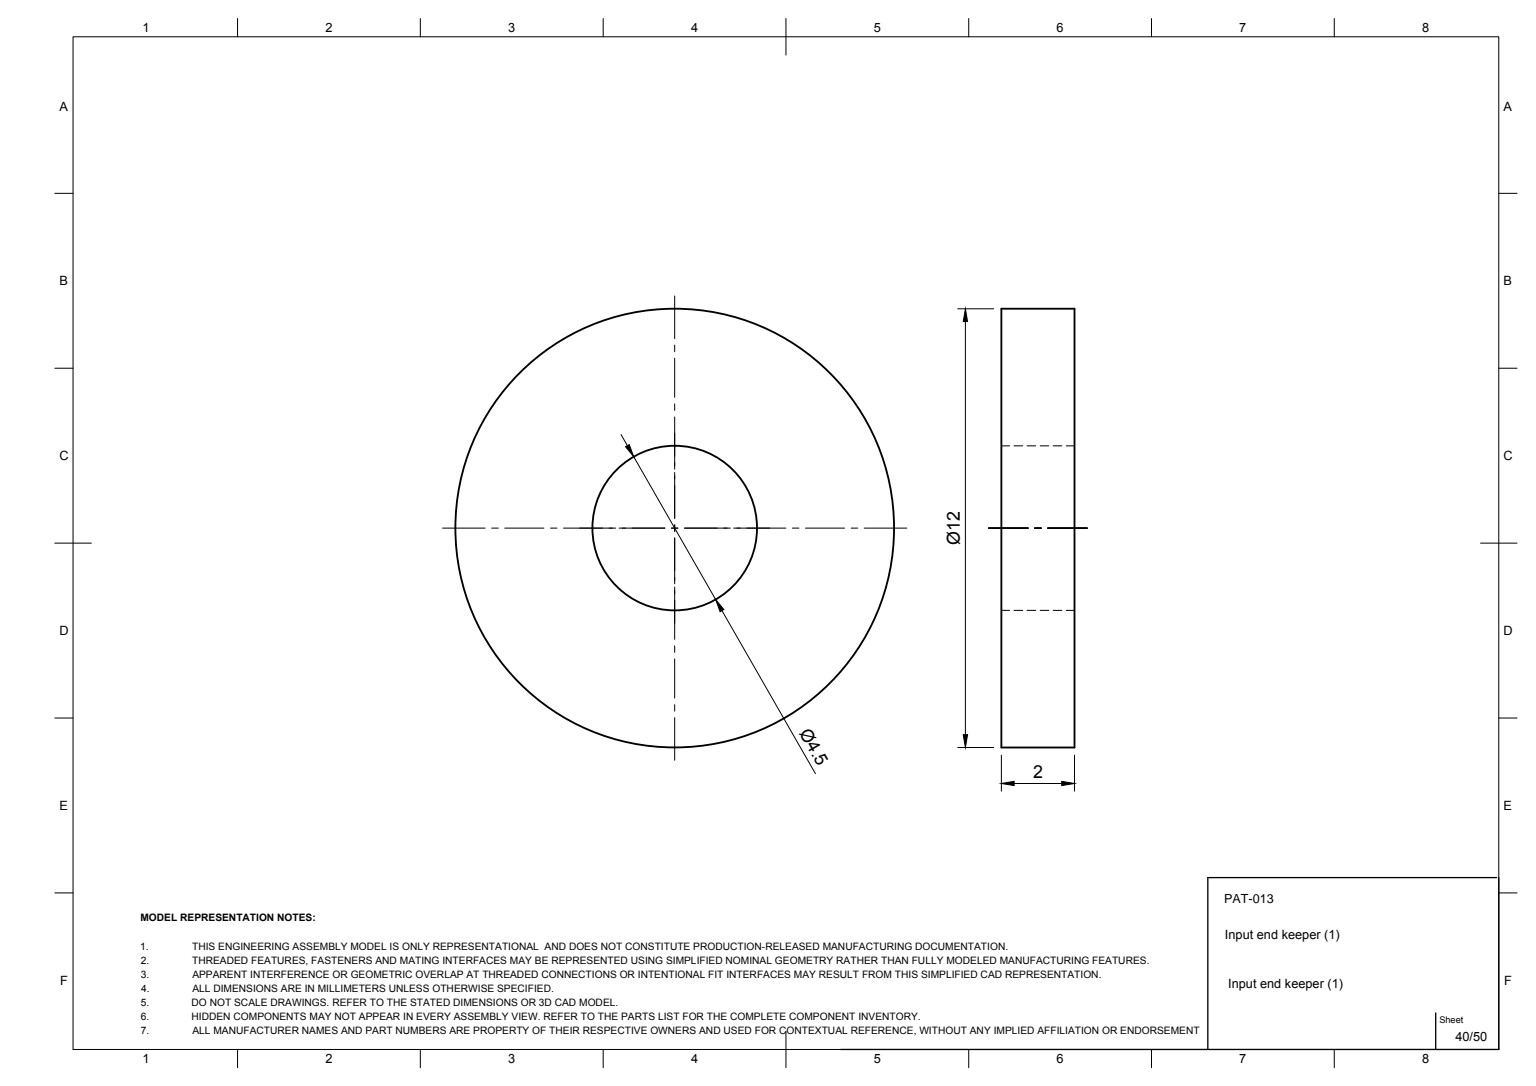
ISO-10303-21;
HEADER;
/* Generated by software containing ST-Developer
 * from STEP Tools, Inc. (www.steptools.com) 
 */

FILE_DESCRIPTION(
/* description */ ('Belt-driven linear axis on 2020 extrusion'),
/* implementation_level */ '2;1');

FILE_NAME(
/* name */ 'Input end keeper (1).step',
/* time_stamp */ '2026-10-28T03:26:09-07:00',
/* author */ (''),
/* organization */ (''),
/* preprocessor_version */ 'ST-DEVELOPER v20.2',
/* originating_system */ 'Autodesk Translation Framework v15.17.0.0',
/* authorisation */ '');

FILE_SCHEMA (('AUTOMOTIVE_DESIGN { 1 0 10303 214 3 1 1 }'));
ENDSEC;

DATA;
#10=MECHANICAL_DESIGN_GEOMETRIC_PRESENTATION_REPRESENTATION('',(#654),#20096);
#552=SHAPE_REPRESENTATION_RELATIONSHIP('SRR','None',#20351,#598);
#598=ADVANCED_BREP_SHAPE_REPRESENTATION('',(#709),#20082);
#654=STYLED_ITEM('',(#20643),#709);
#709=MANIFOLD_SOLID_BREP('Body1',#10968);
#849=FACE_BOUND('',#2432,.T.);
#850=FACE_BOUND('',#2434,.T.);
#1142=PLANE('',#12318);
#1143=PLANE('',#12319);
#1676=FACE_OUTER_BOUND('',#2429,.T.);
#1677=FACE_OUTER_BOUND('',#2430,.T.);
#1678=FACE_OUTER_BOUND('',#2431,.T.);
#1679=FACE_OUTER_BOUND('',#2433,.T.);
#2429=EDGE_LOOP('',(#9121,#9122,#9123,#9124));
#2430=EDGE_LOOP('',(#9125,#9126,#9127,#9128));
#2431=EDGE_LOOP('',(#9129));
#2432=EDGE_LOOP('',(#9130));
#2433=EDGE_LOOP('',(#9131));
#2434=EDGE_LOOP('',(#9132));
#3230=LINE('',#18610,#4087);
#3231=LINE('',#18616,#4088);
#4087=VECTOR('',#14998,0.225000000000001);
#4088=VECTOR('',#15005,0.600000000000001);
#4728=CIRCLE('',#12313,0.225000000000001);
#4729=CIRCLE('',#12314,0.225000000000001);
#4730=CIRCLE('',#12316,0.600000000000001);
#4731=CIRCLE('',#12317,0.600000000000001);
#5523=VERTEX_POINT('',#18607);
#5524=VERTEX_POINT('',#18609);
#5525=VERTEX_POINT('',#18613);
#5526=VERTEX_POINT('',#18615);
#6775=EDGE_CURVE('',#5523,#5523,#4728,.T.);
#6776=EDGE_CURVE('',#5523,#5524,#3230,.T.);
#6777=EDGE_CURVE('',#5524,#5524,#4729,.T.);
#6778=EDGE_CURVE('',#5525,#5525,#4730,.T.);
#6779=EDGE_CURVE('',#5525,#5526,#3231,.T.);
#6780=EDGE_CURVE('',#5526,#5526,#4731,.T.);
#9121=ORIENTED_EDGE('',*,*,#6775,.F.);
#9122=ORIENTED_EDGE('',*,*,#6776,.T.);
#9123=ORIENTED_EDGE('',*,*,#6777,.T.);
#9124=ORIENTED_EDGE('',*,*,#6776,.F.);
#9125=ORIENTED_EDGE('',*,*,#6778,.F.);
#9126=ORIENTED_EDGE('',*,*,#6779,.T.);
#9127=ORIENTED_EDGE('',*,*,#6780,.T.);
#9128=ORIENTED_EDGE('',*,*,#6779,.F.);
#9129=ORIENTED_EDGE('',*,*,#6778,.T.);
#9130=ORIENTED_EDGE('',*,*,#6775,.T.);
#9131=ORIENTED_EDGE('',*,*,#6780,.F.);
#9132=ORIENTED_EDGE('',*,*,#6777,.F.);
#10225=CYLINDRICAL_SURFACE('',#12312,0.225000000000001);
#10226=CYLINDRICAL_SURFACE('',#12315,0.600000000000001);
#10727=ADVANCED_FACE('',(#1676),#10225,.F.);
#10728=ADVANCED_FACE('',(#1677),#10226,.T.);
#10729=ADVANCED_FACE('',(#1678,#849),#1142,.T.);
#10730=ADVANCED_FACE('',(#1679,#850),#1143,.F.);
#10968=CLOSED_SHELL('',(#10727,#10728,#10729,#10730));
#12311=AXIS2_PLACEMENT_3D('',#18605,#14992,#14993);
#12312=AXIS2_PLACEMENT_3D('',#18606,#14994,#14995);
#12313=AXIS2_PLACEMENT_3D('',#18608,#14996,#14997);
#12314=AXIS2_PLACEMENT_3D('',#18611,#14999,#15000);
#12315=AXIS2_PLACEMENT_3D('',#18612,#15001,#15002);
#12316=AXIS2_PLACEMENT_3D('',#18614,#15003,#15004);
#12317=AXIS2_PLACEMENT_3D('',#18617,#15006,#15007);
#12318=AXIS2_PLACEMENT_3D('',#18618,#15008,#15009);
#12319=AXIS2_PLACEMENT_3D('',#18619,#15010,#15011);
#14992=DIRECTION('axis',(0.,0.,1.));
#14993=DIRECTION('refdir',(1.,0.,0.));
#14994=DIRECTION('center_axis',(0.,1.,0.));
#14995=DIRECTION('ref_axis',(1.,0.,0.));
#14996=DIRECTION('center_axis',(0.,-1.,0.));
#14997=DIRECTION('ref_axis',(1.,0.,0.));
#14998=DIRECTION('',(0.,-1.,0.));
#14999=DIRECTION('center_axis',(0.,-1.,0.));
#15000=DIRECTION('ref_axis',(1.,0.,0.));
#15001=DIRECTION('center_axis',(0.,1.,0.));
#15002=DIRECTION('ref_axis',(1.,0.,0.));
#15003=DIRECTION('center_axis',(0.,1.,0.));
#15004=DIRECTION('ref_axis',(1.,0.,0.));
#15005=DIRECTION('',(0.,-1.,0.));
#15006=DIRECTION('center_axis',(0.,1.,0.));
#15007=DIRECTION('ref_axis',(1.,0.,0.));
#15008=DIRECTION('center_axis',(0.,1.,0.));
#15009=DIRECTION('ref_axis',(1.,0.,0.));
#15010=DIRECTION('center_axis',(0.,1.,0.));
#15011=DIRECTION('ref_axis',(1.,0.,0.));
#18605=CARTESIAN_POINT('',(0.,0.,0.));
#18606=CARTESIAN_POINT('Origin',(32.,-5.2,7.));
#18607=CARTESIAN_POINT('',(31.775,-5.,7.));
#18608=CARTESIAN_POINT('Origin',(32.,-5.,7.));
#18609=CARTESIAN_POINT('',(31.775,-5.2,7.));
#18610=CARTESIAN_POINT('',(31.775,-5.2,7.));
#18611=CARTESIAN_POINT('Origin',(32.,-5.2,7.));
#18612=CARTESIAN_POINT('Origin',(32.,-5.2,7.));
#18613=CARTESIAN_POINT('',(31.4,-5.,7.));
#18614=CARTESIAN_POINT('Origin',(32.,-5.,7.));
#18615=CARTESIAN_POINT('',(31.4,-5.2,7.));
#18616=CARTESIAN_POINT('',(31.4,-5.2,7.));
#18617=CARTESIAN_POINT('Origin',(32.,-5.2,7.));
#18618=CARTESIAN_POINT('Origin',(32.,-5.,7.));
#18619=CARTESIAN_POINT('Origin',(32.,-5.2,7.));
#20028=UNCERTAINTY_MEASURE_WITH_UNIT(LENGTH_MEASURE(0.001),#20097,
'DISTANCE_ACCURACY_VALUE',
'Maximum model space distance between geometric entities at asserted c
onnectivities');
#20042=UNCERTAINTY_MEASURE_WITH_UNIT(LENGTH_MEASURE(0.001),#20097,
'DISTANCE_ACCURACY_VALUE',
'Maximum model space distance between geometric entities at asserted c
onnectivities');
#20082=(
GEOMETRIC_REPRESENTATION_CONTEXT(3)
GLOBAL_UNCERTAINTY_ASSIGNED_CONTEXT((#20028))
GLOBAL_UNIT_ASSIGNED_CONTEXT((#20097,#20099,#20100))
REPRESENTATION_CONTEXT('','3D')
);
#20096=(
GEOMETRIC_REPRESENTATION_CONTEXT(3)
GLOBAL_UNCERTAINTY_ASSIGNED_CONTEXT((#20042))
GLOBAL_UNIT_ASSIGNED_CONTEXT((#20097,#20099,#20100))
REPRESENTATION_CONTEXT('','3D')
);
#20097=(
LENGTH_UNIT()
NAMED_UNIT(*)
SI_UNIT(.CENTI.,.METRE.)
);
#20099=(
NAMED_UNIT(*)
PLANE_ANGLE_UNIT()
SI_UNIT($,.RADIAN.)
);
#20100=(
NAMED_UNIT(*)
SI_UNIT($,.STERADIAN.)
SOLID_ANGLE_UNIT()
);
#20140=SHAPE_DEFINITION_REPRESENTATION(#20198,#20351);
#20198=PRODUCT_DEFINITION_SHAPE('',$,#20405);
#20351=SHAPE_REPRESENTATION('',(#12311),#20082);
#20365=PRODUCT_DEFINITION_CONTEXT('part definition',#20526,'design');
#20405=PRODUCT_DEFINITION('Input end keeper (1)','Input end keeper (1)',#20458,
#20365);
#20458=PRODUCT_DEFINITION_FORMATION('',$,#20567);
#20526=APPLICATION_CONTEXT(
'Core Data for Automotive Mechanical Design Process');
#20527=PRODUCT_CONTEXT('part definition',#20526,'mechanical');
#20567=PRODUCT('Input end keeper (1)','Input end keeper (1)',
'Input end keeper (1)',(#20527));
#20637=COLOUR_RGB('Sky Blue',0.24,0.69,0.87);
#20638=FILL_AREA_STYLE_COLOUR('',#20637);
#20639=FILL_AREA_STYLE('',(#20638));
#20640=SURFACE_STYLE_FILL_AREA(#20639);
#20641=SURFACE_SIDE_STYLE('',(#20640));
#20642=SURFACE_STYLE_USAGE(.BOTH.,#20641);
#20643=PRESENTATION_STYLE_ASSIGNMENT((#20642));
ENDSEC;
END-ISO-10303-21;
